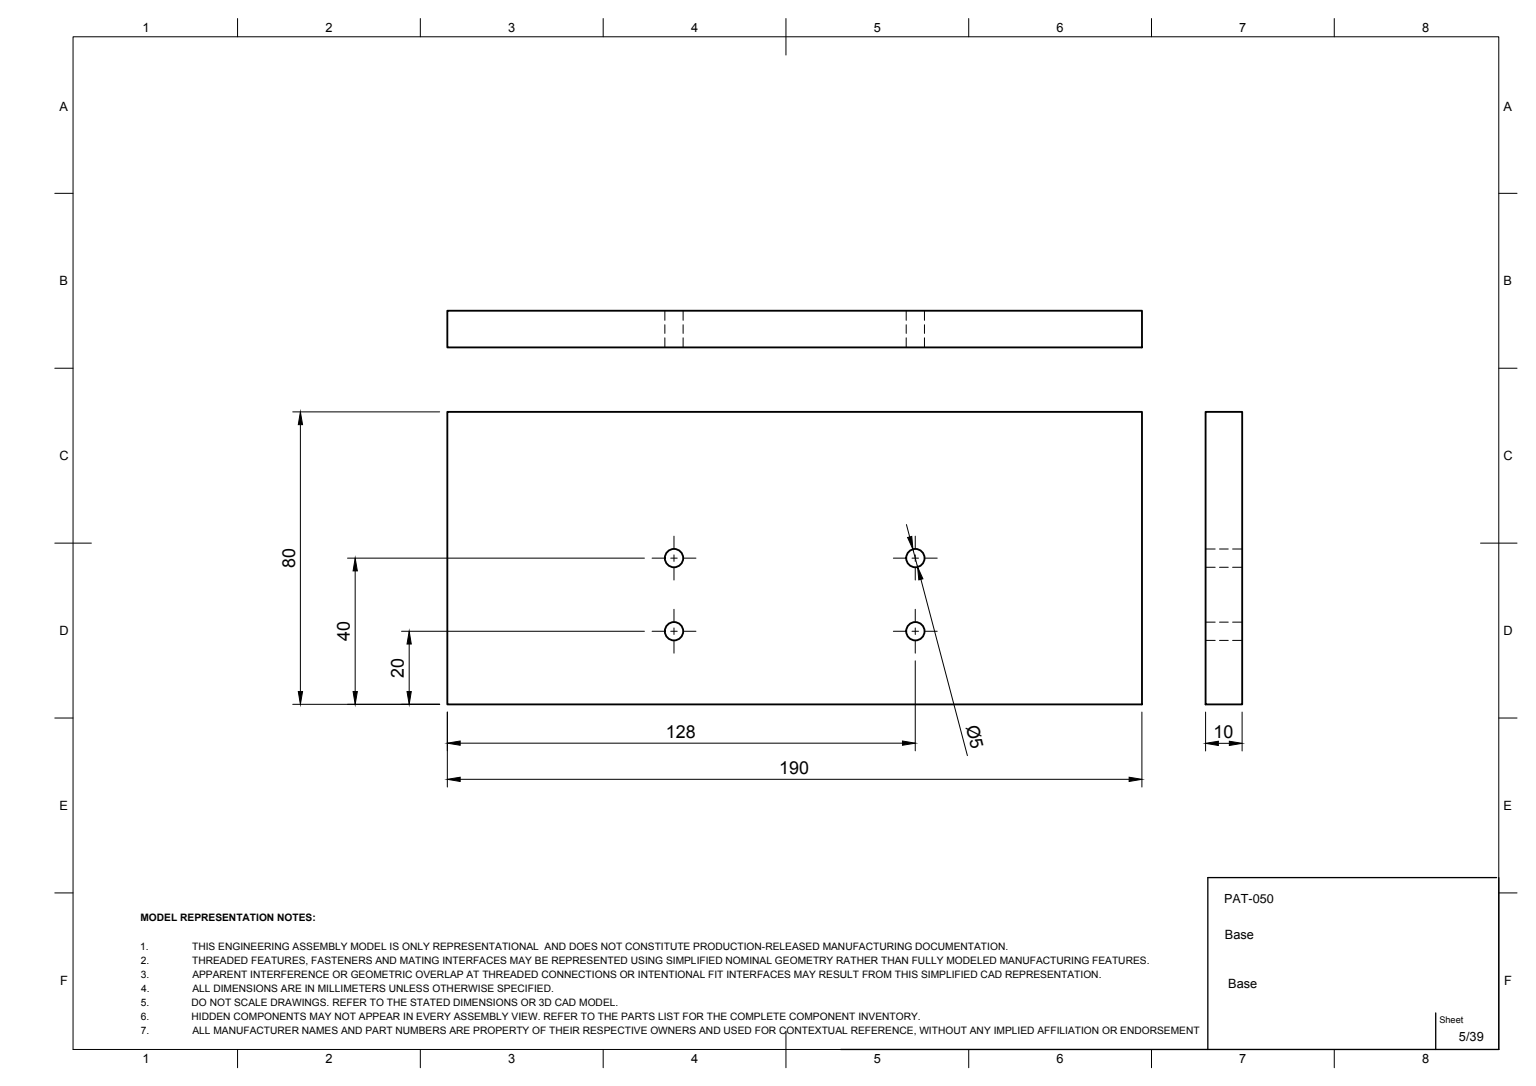
ISO-10303-21;
HEADER;
/* Generated by software containing ST-Developer
 * from STEP Tools, Inc. (www.steptools.com) 
 */

FILE_DESCRIPTION(
/* description */ ('Hand wheel with handle and shaft collar'),
/* implementation_level */ '2;1');

FILE_NAME(
/* name */ 'Base.step',
/* time_stamp */ '2026-10-28T03:23:19-07:00',
/* author */ (''),
/* organization */ (''),
/* preprocessor_version */ 'ST-DEVELOPER v20.2',
/* originating_system */ 'Autodesk Translation Framework v15.17.0.0',
/* authorisation */ '');

FILE_SCHEMA (('AUTOMOTIVE_DESIGN { 1 0 10303 214 3 1 1 }'));
ENDSEC;

DATA;
#10=MECHANICAL_DESIGN_GEOMETRIC_PRESENTATION_REPRESENTATION('',(#395),#10510);
#331=SHAPE_REPRESENTATION_RELATIONSHIP('SRR','None',#10647,#363);
#363=ADVANCED_BREP_SHAPE_REPRESENTATION('',(#442),#10474);
#395=STYLED_ITEM('',(#10887),#442);
#442=MANIFOLD_SOLID_BREP('Body1',#5294);
#486=FACE_BOUND('',#1091,.T.);
#487=FACE_BOUND('',#1092,.T.);
#488=FACE_BOUND('',#1093,.T.);
#489=FACE_BOUND('',#1094,.T.);
#490=FACE_BOUND('',#1096,.T.);
#491=FACE_BOUND('',#1097,.T.);
#492=FACE_BOUND('',#1098,.T.);
#493=FACE_BOUND('',#1099,.T.);
#598=PLANE('',#5712);
#599=PLANE('',#5713);
#600=PLANE('',#5714);
#601=PLANE('',#5715);
#602=PLANE('',#5716);
#603=PLANE('',#5717);
#763=FACE_OUTER_BOUND('',#1082,.T.);
#764=FACE_OUTER_BOUND('',#1083,.T.);
#765=FACE_OUTER_BOUND('',#1084,.T.);
#766=FACE_OUTER_BOUND('',#1085,.T.);
#767=FACE_OUTER_BOUND('',#1086,.T.);
#768=FACE_OUTER_BOUND('',#1087,.T.);
#769=FACE_OUTER_BOUND('',#1088,.T.);
#770=FACE_OUTER_BOUND('',#1089,.T.);
#771=FACE_OUTER_BOUND('',#1090,.T.);
#772=FACE_OUTER_BOUND('',#1095,.T.);
#1082=EDGE_LOOP('',(#3557,#3558,#3559,#3560));
#1083=EDGE_LOOP('',(#3561,#3562,#3563,#3564));
#1084=EDGE_LOOP('',(#3565,#3566,#3567,#3568));
#1085=EDGE_LOOP('',(#3569,#3570,#3571,#3572));
#1086=EDGE_LOOP('',(#3573,#3574,#3575,#3576));
#1087=EDGE_LOOP('',(#3577,#3578,#3579,#3580));
#1088=EDGE_LOOP('',(#3581,#3582,#3583,#3584));
#1089=EDGE_LOOP('',(#3585,#3586,#3587,#3588));
#1090=EDGE_LOOP('',(#3589,#3590,#3591,#3592));
#1091=EDGE_LOOP('',(#3593));
#1092=EDGE_LOOP('',(#3594));
#1093=EDGE_LOOP('',(#3595));
#1094=EDGE_LOOP('',(#3596));
#1095=EDGE_LOOP('',(#3597,#3598,#3599,#3600));
#1096=EDGE_LOOP('',(#3601));
#1097=EDGE_LOOP('',(#3602));
#1098=EDGE_LOOP('',(#3603));
#1099=EDGE_LOOP('',(#3604));
#1513=LINE('',#8180,#1823);
#1514=LINE('',#8186,#1824);
#1515=LINE('',#8192,#1825);
#1516=LINE('',#8198,#1826);
#1517=LINE('',#8203,#1827);
#1518=LINE('',#8205,#1828);
#1519=LINE('',#8207,#1829);
#1520=LINE('',#8208,#1830);
#1521=LINE('',#8211,#1831);
#1522=LINE('',#8213,#1832);
#1523=LINE('',#8214,#1833);
#1524=LINE('',#8217,#1834);
#1525=LINE('',#8219,#1835);
#1526=LINE('',#8220,#1836);
#1527=LINE('',#8222,#1837);
#1528=LINE('',#8223,#1838);
#1823=VECTOR('',#6429,0.25);
#1824=VECTOR('',#6436,0.25);
#1825=VECTOR('',#6443,0.25);
#1826=VECTOR('',#6450,0.25);
#1827=VECTOR('',#6455,1.);
#1828=VECTOR('',#6456,1.);
#1829=VECTOR('',#6457,1.);
#1830=VECTOR('',#6458,1.);
#1831=VECTOR('',#6461,1.);
#1832=VECTOR('',#6462,1.);
#1833=VECTOR('',#6463,1.);
#1834=VECTOR('',#6466,1.);
#1835=VECTOR('',#6467,1.);
#1836=VECTOR('',#6468,1.);
#1837=VECTOR('',#6471,1.);
#1838=VECTOR('',#6472,1.);
#2133=CIRCLE('',#5701,0.25);
#2134=CIRCLE('',#5702,0.25);
#2135=CIRCLE('',#5704,0.25);
#2136=CIRCLE('',#5705,0.25);
#2137=CIRCLE('',#5707,0.25);
#2138=CIRCLE('',#5708,0.25);
#2139=CIRCLE('',#5710,0.25);
#2140=CIRCLE('',#5711,0.25);
#2444=VERTEX_POINT('',#8177);
#2445=VERTEX_POINT('',#8179);
#2446=VERTEX_POINT('',#8183);
#2447=VERTEX_POINT('',#8185);
#2448=VERTEX_POINT('',#8189);
#2449=VERTEX_POINT('',#8191);
#2450=VERTEX_POINT('',#8195);
#2451=VERTEX_POINT('',#8197);
#2452=VERTEX_POINT('',#8201);
#2453=VERTEX_POINT('',#8202);
#2454=VERTEX_POINT('',#8204);
#2455=VERTEX_POINT('',#8206);
#2456=VERTEX_POINT('',#8210);
#2457=VERTEX_POINT('',#8212);
#2458=VERTEX_POINT('',#8216);
#2459=VERTEX_POINT('',#8218);
#2896=EDGE_CURVE('',#2444,#2444,#2133,.T.);
#2897=EDGE_CURVE('',#2444,#2445,#1513,.T.);
#2898=EDGE_CURVE('',#2445,#2445,#2134,.T.);
#2899=EDGE_CURVE('',#2446,#2446,#2135,.T.);
#2900=EDGE_CURVE('',#2446,#2447,#1514,.T.);
#2901=EDGE_CURVE('',#2447,#2447,#2136,.T.);
#2902=EDGE_CURVE('',#2448,#2448,#2137,.T.);
#2903=EDGE_CURVE('',#2448,#2449,#1515,.T.);
#2904=EDGE_CURVE('',#2449,#2449,#2138,.T.);
#2905=EDGE_CURVE('',#2450,#2450,#2139,.T.);
#2906=EDGE_CURVE('',#2450,#2451,#1516,.T.);
#2907=EDGE_CURVE('',#2451,#2451,#2140,.T.);
#2908=EDGE_CURVE('',#2452,#2453,#1517,.T.);
#2909=EDGE_CURVE('',#2453,#2454,#1518,.T.);
#2910=EDGE_CURVE('',#2455,#2454,#1519,.T.);
#2911=EDGE_CURVE('',#2452,#2455,#1520,.T.);
#2912=EDGE_CURVE('',#2456,#2452,#1521,.T.);
#2913=EDGE_CURVE('',#2457,#2455,#1522,.T.);
#2914=EDGE_CURVE('',#2456,#2457,#1523,.T.);
#2915=EDGE_CURVE('',#2458,#2456,#1524,.T.);
#2916=EDGE_CURVE('',#2459,#2457,#1525,.T.);
#2917=EDGE_CURVE('',#2458,#2459,#1526,.T.);
#2918=EDGE_CURVE('',#2453,#2458,#1527,.T.);
#2919=EDGE_CURVE('',#2454,#2459,#1528,.T.);
#3557=ORIENTED_EDGE('',*,*,#2896,.F.);
#3558=ORIENTED_EDGE('',*,*,#2897,.T.);
#3559=ORIENTED_EDGE('',*,*,#2898,.F.);
#3560=ORIENTED_EDGE('',*,*,#2897,.F.);
#3561=ORIENTED_EDGE('',*,*,#2899,.F.);
#3562=ORIENTED_EDGE('',*,*,#2900,.T.);
#3563=ORIENTED_EDGE('',*,*,#2901,.F.);
#3564=ORIENTED_EDGE('',*,*,#2900,.F.);
#3565=ORIENTED_EDGE('',*,*,#2902,.F.);
#3566=ORIENTED_EDGE('',*,*,#2903,.T.);
#3567=ORIENTED_EDGE('',*,*,#2904,.F.);
#3568=ORIENTED_EDGE('',*,*,#2903,.F.);
#3569=ORIENTED_EDGE('',*,*,#2905,.F.);
#3570=ORIENTED_EDGE('',*,*,#2906,.T.);
#3571=ORIENTED_EDGE('',*,*,#2907,.F.);
#3572=ORIENTED_EDGE('',*,*,#2906,.F.);
#3573=ORIENTED_EDGE('',*,*,#2908,.T.);
#3574=ORIENTED_EDGE('',*,*,#2909,.T.);
#3575=ORIENTED_EDGE('',*,*,#2910,.F.);
#3576=ORIENTED_EDGE('',*,*,#2911,.F.);
#3577=ORIENTED_EDGE('',*,*,#2912,.T.);
#3578=ORIENTED_EDGE('',*,*,#2911,.T.);
#3579=ORIENTED_EDGE('',*,*,#2913,.F.);
#3580=ORIENTED_EDGE('',*,*,#2914,.F.);
#3581=ORIENTED_EDGE('',*,*,#2915,.T.);
#3582=ORIENTED_EDGE('',*,*,#2914,.T.);
#3583=ORIENTED_EDGE('',*,*,#2916,.F.);
#3584=ORIENTED_EDGE('',*,*,#2917,.F.);
#3585=ORIENTED_EDGE('',*,*,#2918,.T.);
#3586=ORIENTED_EDGE('',*,*,#2917,.T.);
#3587=ORIENTED_EDGE('',*,*,#2919,.F.);
#3588=ORIENTED_EDGE('',*,*,#2909,.F.);
#3589=ORIENTED_EDGE('',*,*,#2919,.T.);
#3590=ORIENTED_EDGE('',*,*,#2916,.T.);
#3591=ORIENTED_EDGE('',*,*,#2913,.T.);
#3592=ORIENTED_EDGE('',*,*,#2910,.T.);
#3593=ORIENTED_EDGE('',*,*,#2898,.T.);
#3594=ORIENTED_EDGE('',*,*,#2901,.T.);
#3595=ORIENTED_EDGE('',*,*,#2904,.T.);
#3596=ORIENTED_EDGE('',*,*,#2907,.T.);
#3597=ORIENTED_EDGE('',*,*,#2918,.F.);
#3598=ORIENTED_EDGE('',*,*,#2908,.F.);
#3599=ORIENTED_EDGE('',*,*,#2912,.F.);
#3600=ORIENTED_EDGE('',*,*,#2915,.F.);
#3601=ORIENTED_EDGE('',*,*,#2896,.T.);
#3602=ORIENTED_EDGE('',*,*,#2899,.T.);
#3603=ORIENTED_EDGE('',*,*,#2902,.T.);
#3604=ORIENTED_EDGE('',*,*,#2905,.T.);
#4879=CYLINDRICAL_SURFACE('',#5700,0.25);
#4880=CYLINDRICAL_SURFACE('',#5703,0.25);
#4881=CYLINDRICAL_SURFACE('',#5706,0.25);
#4882=CYLINDRICAL_SURFACE('',#5709,0.25);
#4975=ADVANCED_FACE('',(#763),#4879,.F.);
#4976=ADVANCED_FACE('',(#764),#4880,.F.);
#4977=ADVANCED_FACE('',(#765),#4881,.F.);
#4978=ADVANCED_FACE('',(#766),#4882,.F.);
#4979=ADVANCED_FACE('',(#767),#598,.T.);
#4980=ADVANCED_FACE('',(#768),#599,.T.);
#4981=ADVANCED_FACE('',(#769),#600,.T.);
#4982=ADVANCED_FACE('',(#770),#601,.T.);
#4983=ADVANCED_FACE('',(#771,#486,#487,#488,#489),#602,.T.);
#4984=ADVANCED_FACE('',(#772,#490,#491,#492,#493),#603,.F.);
#5294=CLOSED_SHELL('',(#4975,#4976,#4977,#4978,#4979,#4980,#4981,#4982,
#4983,#4984));
#5699=AXIS2_PLACEMENT_3D('',#8175,#6423,#6424);
#5700=AXIS2_PLACEMENT_3D('',#8176,#6425,#6426);
#5701=AXIS2_PLACEMENT_3D('',#8178,#6427,#6428);
#5702=AXIS2_PLACEMENT_3D('',#8181,#6430,#6431);
#5703=AXIS2_PLACEMENT_3D('',#8182,#6432,#6433);
#5704=AXIS2_PLACEMENT_3D('',#8184,#6434,#6435);
#5705=AXIS2_PLACEMENT_3D('',#8187,#6437,#6438);
#5706=AXIS2_PLACEMENT_3D('',#8188,#6439,#6440);
#5707=AXIS2_PLACEMENT_3D('',#8190,#6441,#6442);
#5708=AXIS2_PLACEMENT_3D('',#8193,#6444,#6445);
#5709=AXIS2_PLACEMENT_3D('',#8194,#6446,#6447);
#5710=AXIS2_PLACEMENT_3D('',#8196,#6448,#6449);
#5711=AXIS2_PLACEMENT_3D('',#8199,#6451,#6452);
#5712=AXIS2_PLACEMENT_3D('',#8200,#6453,#6454);
#5713=AXIS2_PLACEMENT_3D('',#8209,#6459,#6460);
#5714=AXIS2_PLACEMENT_3D('',#8215,#6464,#6465);
#5715=AXIS2_PLACEMENT_3D('',#8221,#6469,#6470);
#5716=AXIS2_PLACEMENT_3D('',#8224,#6473,#6474);
#5717=AXIS2_PLACEMENT_3D('',#8225,#6475,#6476);
#6423=DIRECTION('axis',(0.,0.,1.));
#6424=DIRECTION('refdir',(1.,0.,0.));
#6425=DIRECTION('center_axis',(0.,0.,1.));
#6426=DIRECTION('ref_axis',(1.,0.,0.));
#6427=DIRECTION('center_axis',(0.,0.,1.));
#6428=DIRECTION('ref_axis',(1.,0.,0.));
#6429=DIRECTION('',(0.,0.,1.));
#6430=DIRECTION('center_axis',(0.,0.,-1.));
#6431=DIRECTION('ref_axis',(1.,0.,0.));
#6432=DIRECTION('center_axis',(0.,0.,1.));
#6433=DIRECTION('ref_axis',(1.,0.,0.));
#6434=DIRECTION('center_axis',(0.,0.,1.));
#6435=DIRECTION('ref_axis',(1.,0.,0.));
#6436=DIRECTION('',(0.,0.,1.));
#6437=DIRECTION('center_axis',(0.,0.,-1.));
#6438=DIRECTION('ref_axis',(1.,0.,0.));
#6439=DIRECTION('center_axis',(0.,0.,1.));
#6440=DIRECTION('ref_axis',(1.,0.,0.));
#6441=DIRECTION('center_axis',(0.,0.,1.));
#6442=DIRECTION('ref_axis',(1.,0.,0.));
#6443=DIRECTION('',(0.,0.,1.));
#6444=DIRECTION('center_axis',(0.,0.,-1.));
#6445=DIRECTION('ref_axis',(1.,0.,0.));
#6446=DIRECTION('center_axis',(0.,0.,1.));
#6447=DIRECTION('ref_axis',(1.,0.,0.));
#6448=DIRECTION('center_axis',(0.,0.,1.));
#6449=DIRECTION('ref_axis',(1.,0.,0.));
#6450=DIRECTION('',(0.,0.,1.));
#6451=DIRECTION('center_axis',(0.,0.,-1.));
#6452=DIRECTION('ref_axis',(1.,0.,0.));
#6453=DIRECTION('center_axis',(0.,1.,0.));
#6454=DIRECTION('ref_axis',(-1.,0.,0.));
#6455=DIRECTION('',(-1.,0.,0.));
#6456=DIRECTION('',(0.,0.,1.));
#6457=DIRECTION('',(-1.,0.,0.));
#6458=DIRECTION('',(0.,0.,1.));
#6459=DIRECTION('center_axis',(1.,0.,0.));
#6460=DIRECTION('ref_axis',(0.,1.,0.));
#6461=DIRECTION('',(0.,1.,0.));
#6462=DIRECTION('',(0.,1.,0.));
#6463=DIRECTION('',(0.,0.,1.));
#6464=DIRECTION('center_axis',(0.,-1.,0.));
#6465=DIRECTION('ref_axis',(1.,0.,0.));
#6466=DIRECTION('',(1.,0.,0.));
#6467=DIRECTION('',(1.,0.,0.));
#6468=DIRECTION('',(0.,0.,1.));
#6469=DIRECTION('center_axis',(-1.,0.,0.));
#6470=DIRECTION('ref_axis',(0.,-1.,0.));
#6471=DIRECTION('',(0.,-1.,0.));
#6472=DIRECTION('',(0.,-1.,0.));
#6473=DIRECTION('center_axis',(0.,0.,1.));
#6474=DIRECTION('ref_axis',(1.,0.,0.));
#6475=DIRECTION('center_axis',(0.,0.,1.));
#6476=DIRECTION('ref_axis',(1.,0.,0.));
#8175=CARTESIAN_POINT('',(0.,0.,0.));
#8176=CARTESIAN_POINT('Origin',(3.3,1.,-0.1));
#8177=CARTESIAN_POINT('',(3.05,1.,0.));
#8178=CARTESIAN_POINT('Origin',(3.3,1.,0.));
#8179=CARTESIAN_POINT('',(3.05,1.,1.));
#8180=CARTESIAN_POINT('',(3.05,1.,-0.1));
#8181=CARTESIAN_POINT('Origin',(3.3,1.,1.));
#8182=CARTESIAN_POINT('Origin',(-3.3,3.,-0.1));
#8183=CARTESIAN_POINT('',(-3.55,3.,0.));
#8184=CARTESIAN_POINT('Origin',(-3.3,3.,0.));
#8185=CARTESIAN_POINT('',(-3.55,3.,1.));
#8186=CARTESIAN_POINT('',(-3.55,3.,-0.1));
#8187=CARTESIAN_POINT('Origin',(-3.3,3.,1.));
#8188=CARTESIAN_POINT('Origin',(-3.3,1.,-0.1));
#8189=CARTESIAN_POINT('',(-3.55,1.,0.));
#8190=CARTESIAN_POINT('Origin',(-3.3,1.,0.));
#8191=CARTESIAN_POINT('',(-3.55,1.,1.));
#8192=CARTESIAN_POINT('',(-3.55,1.,-0.1));
#8193=CARTESIAN_POINT('Origin',(-3.3,1.,1.));
#8194=CARTESIAN_POINT('Origin',(3.3,3.,-0.1));
#8195=CARTESIAN_POINT('',(3.05,3.,0.));
#8196=CARTESIAN_POINT('Origin',(3.3,3.,0.));
#8197=CARTESIAN_POINT('',(3.05,3.,1.));
#8198=CARTESIAN_POINT('',(3.05,3.,-0.1));
#8199=CARTESIAN_POINT('Origin',(3.3,3.,1.));
#8200=CARTESIAN_POINT('Origin',(9.5,7.,0.));
#8201=CARTESIAN_POINT('',(9.5,7.,0.));
#8202=CARTESIAN_POINT('',(-9.5,7.,0.));
#8203=CARTESIAN_POINT('',(9.5,7.,0.));
#8204=CARTESIAN_POINT('',(-9.5,7.,1.));
#8205=CARTESIAN_POINT('',(-9.5,7.,0.));
#8206=CARTESIAN_POINT('',(9.5,7.,1.));
#8207=CARTESIAN_POINT('',(9.5,7.,1.));
#8208=CARTESIAN_POINT('',(9.5,7.,0.));
#8209=CARTESIAN_POINT('Origin',(9.5,-1.,0.));
#8210=CARTESIAN_POINT('',(9.5,-1.,0.));
#8211=CARTESIAN_POINT('',(9.5,-1.,0.));
#8212=CARTESIAN_POINT('',(9.5,-1.,1.));
#8213=CARTESIAN_POINT('',(9.5,-1.,1.));
#8214=CARTESIAN_POINT('',(9.5,-1.,0.));
#8215=CARTESIAN_POINT('Origin',(-9.5,-1.,0.));
#8216=CARTESIAN_POINT('',(-9.5,-1.,0.));
#8217=CARTESIAN_POINT('',(-9.5,-1.,0.));
#8218=CARTESIAN_POINT('',(-9.5,-1.,1.));
#8219=CARTESIAN_POINT('',(-9.5,-1.,1.));
#8220=CARTESIAN_POINT('',(-9.5,-1.,0.));
#8221=CARTESIAN_POINT('Origin',(-9.5,7.,0.));
#8222=CARTESIAN_POINT('',(-9.5,7.,0.));
#8223=CARTESIAN_POINT('',(-9.5,7.,1.));
#8224=CARTESIAN_POINT('Origin',(0.,3.,1.));
#8225=CARTESIAN_POINT('Origin',(0.,3.,0.));
#10435=UNCERTAINTY_MEASURE_WITH_UNIT(LENGTH_MEASURE(0.001),#10511,
'DISTANCE_ACCURACY_VALUE',
'Maximum model space distance between geometric entities at asserted c
onnectivities');
#10471=UNCERTAINTY_MEASURE_WITH_UNIT(LENGTH_MEASURE(0.001),#10511,
'DISTANCE_ACCURACY_VALUE',
'Maximum model space distance between geometric entities at asserted c
onnectivities');
#10474=(
GEOMETRIC_REPRESENTATION_CONTEXT(3)
GLOBAL_UNCERTAINTY_ASSIGNED_CONTEXT((#10435))
GLOBAL_UNIT_ASSIGNED_CONTEXT((#10511,#10513,#10514))
REPRESENTATION_CONTEXT('','3D')
);
#10510=(
GEOMETRIC_REPRESENTATION_CONTEXT(3)
GLOBAL_UNCERTAINTY_ASSIGNED_CONTEXT((#10471))
GLOBAL_UNIT_ASSIGNED_CONTEXT((#10511,#10513,#10514))
REPRESENTATION_CONTEXT('','3D')
);
#10511=(
LENGTH_UNIT()
NAMED_UNIT(*)
SI_UNIT(.CENTI.,.METRE.)
);
#10513=(
NAMED_UNIT(*)
PLANE_ANGLE_UNIT()
SI_UNIT($,.RADIAN.)
);
#10514=(
NAMED_UNIT(*)
SI_UNIT($,.STERADIAN.)
SOLID_ANGLE_UNIT()
);
#10517=SHAPE_DEFINITION_REPRESENTATION(#10555,#10647);
#10555=PRODUCT_DEFINITION_SHAPE('',$,#10686);
#10647=SHAPE_REPRESENTATION('',(#5699),#10474);
#10683=PRODUCT_DEFINITION_CONTEXT('part definition',#10799,'design');
#10686=PRODUCT_DEFINITION('Base','Base',#10724,#10683);
#10724=PRODUCT_DEFINITION_FORMATION('',$,#10803);
#10799=APPLICATION_CONTEXT(
'Core Data for Automotive Mechanical Design Process');
#10800=PRODUCT_CONTEXT('part definition',#10799,'mechanical');
#10803=PRODUCT('Base','Base','Base',(#10800));
#10881=COLOUR_RGB('Dark Blue',0.08,0.2,0.34);
#10882=FILL_AREA_STYLE_COLOUR('',#10881);
#10883=FILL_AREA_STYLE('',(#10882));
#10884=SURFACE_STYLE_FILL_AREA(#10883);
#10885=SURFACE_SIDE_STYLE('',(#10884));
#10886=SURFACE_STYLE_USAGE(.BOTH.,#10885);
#10887=PRESENTATION_STYLE_ASSIGNMENT((#10886));
ENDSEC;
END-ISO-10303-21;
